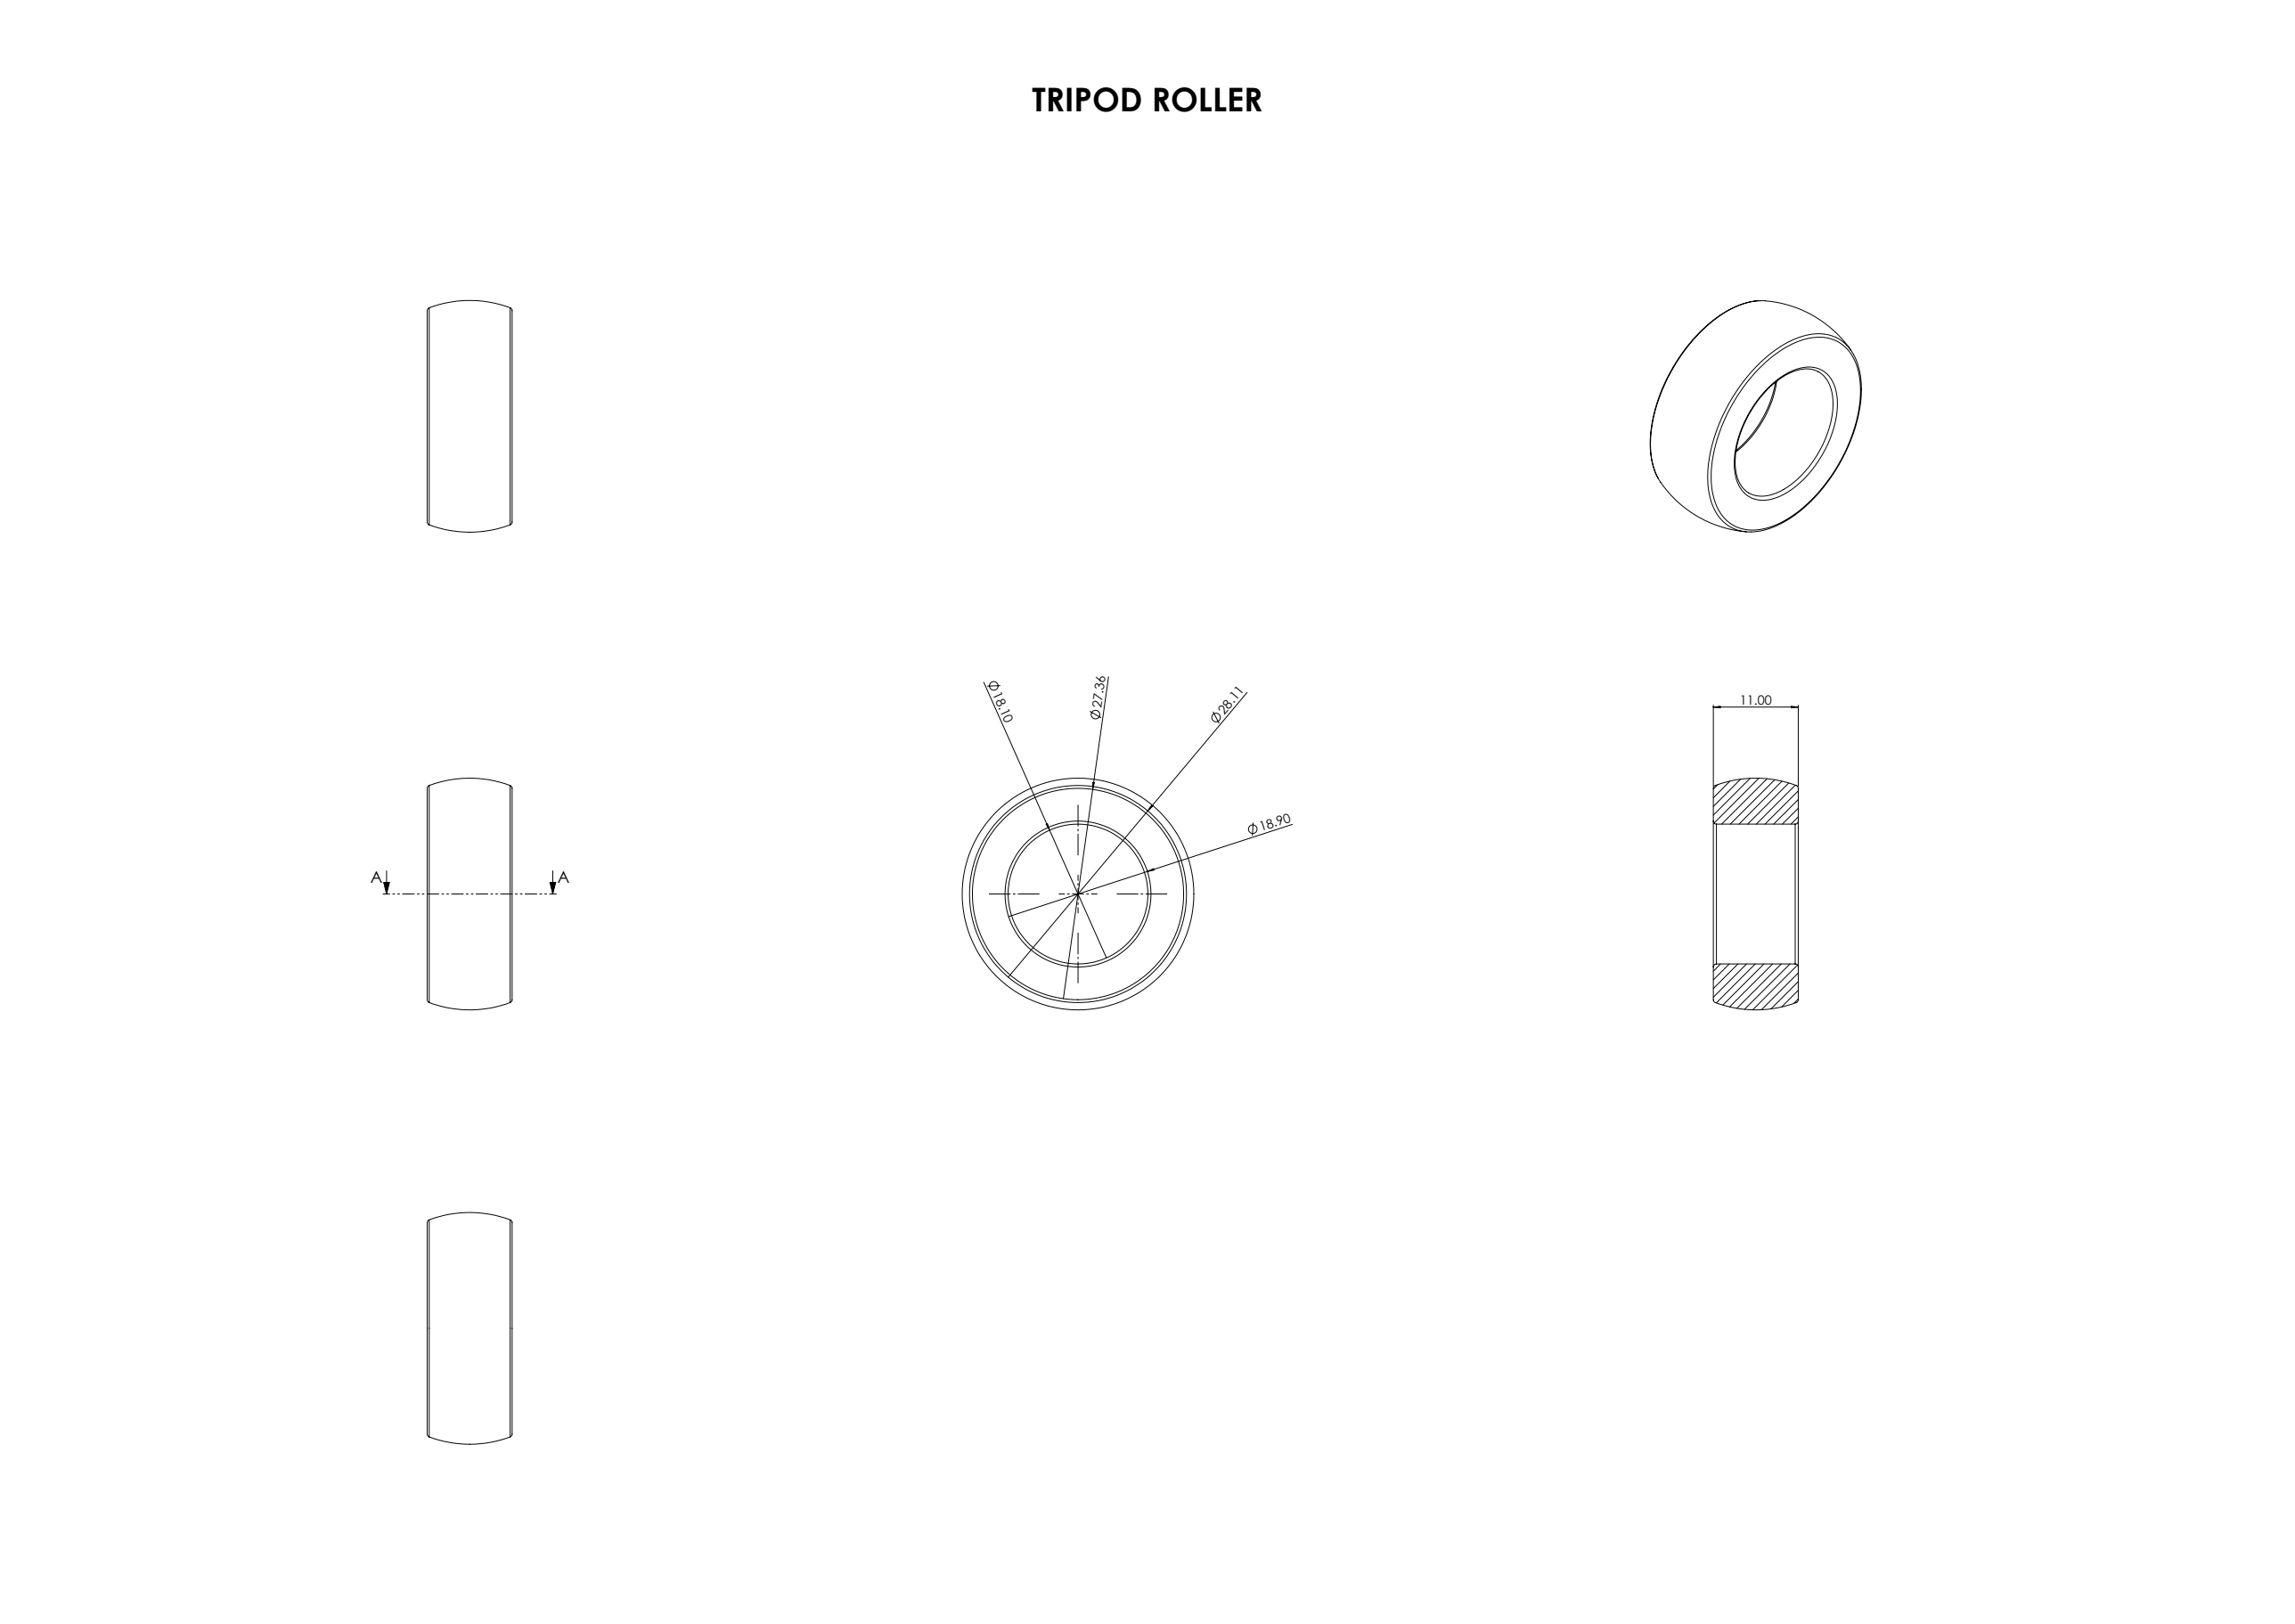
ISO-10303-21;
HEADER;
/* Generated by software containing ST-Developer
 * from STEP Tools, Inc. (www.steptools.com) 
 */

FILE_DESCRIPTION(
/* description */ (''),
/* implementation_level */ '2;1');

FILE_NAME(
/* name */ '15_Tripod_Roller.step',
/* time_stamp */ '2026-10-11T12:57:03-07:00',
/* author */ (''),
/* organization */ (''),
/* preprocessor_version */ 'ST-DEVELOPER v20.2',
/* originating_system */ 'Autodesk Translation Framework v15.15.0.0',
/* authorisation */ '');

FILE_SCHEMA (('AUTOMOTIVE_DESIGN { 1 0 10303 214 3 1 1 }'));
ENDSEC;

DATA;
#10=MECHANICAL_DESIGN_GEOMETRIC_PRESENTATION_REPRESENTATION('',(#270),#90374);
#236=SHAPE_REPRESENTATION_RELATIONSHIP('SRR','None',#90455,#253);
#253=ADVANCED_BREP_SHAPE_REPRESENTATION('',(#287),#90371);
#270=STYLED_ITEM('',(#90673),#287);
#287=MANIFOLD_SOLID_BREP('Body1',#40359);
#573=SPHERICAL_SURFACE('',#45209,15.);
#1031=TOROIDAL_SURFACE('',#45202,13.6802777749576,0.4);
#1032=TOROIDAL_SURFACE('',#45213,9.45,0.4);
#1033=TOROIDAL_SURFACE('',#45220,9.45,0.4);
#1034=TOROIDAL_SURFACE('',#45225,13.6802777749576,0.4);
#1110=FACE_BOUND('',#6986,.T.);
#1111=FACE_BOUND('',#6988,.T.);
#1112=FACE_BOUND('',#6993,.T.);
#1819=PLANE('',#45207);
#1820=PLANE('',#45223);
#4517=FACE_OUTER_BOUND('',#6984,.T.);
#4518=FACE_OUTER_BOUND('',#6985,.T.);
#4519=FACE_OUTER_BOUND('',#6987,.T.);
#4520=FACE_OUTER_BOUND('',#6989,.T.);
#4521=FACE_OUTER_BOUND('',#6990,.T.);
#4522=FACE_OUTER_BOUND('',#6991,.T.);
#4523=FACE_OUTER_BOUND('',#6992,.T.);
#4524=FACE_OUTER_BOUND('',#6994,.T.);
#6984=EDGE_LOOP('',(#37119,#37120,#37121,#37122,#37123));
#6985=EDGE_LOOP('',(#37124));
#6986=EDGE_LOOP('',(#37125));
#6987=EDGE_LOOP('',(#37126,#37127,#37128,#37129,#37130,#37131));
#6988=EDGE_LOOP('',(#37132));
#6989=EDGE_LOOP('',(#37133,#37134,#37135,#37136,#37137));
#6990=EDGE_LOOP('',(#37138,#37139,#37140,#37141,#37142,#37143));
#6991=EDGE_LOOP('',(#37144,#37145,#37146,#37147,#37148));
#6992=EDGE_LOOP('',(#37149));
#6993=EDGE_LOOP('',(#37150));
#6994=EDGE_LOOP('',(#37151,#37152,#37153,#37154));
#9382=CIRCLE('',#45203,14.0550799057784);
#9383=CIRCLE('',#45204,14.0550799057784);
#9384=CIRCLE('',#45205,0.4);
#9385=CIRCLE('',#45206,13.6802777749576);
#9386=CIRCLE('',#45208,9.45);
#9387=CIRCLE('',#45210,15.);
#9388=CIRCLE('',#45211,15.);
#9389=CIRCLE('',#45212,14.0550799057784);
#9390=CIRCLE('',#45214,0.4);
#9391=CIRCLE('',#45215,9.05);
#9392=CIRCLE('',#45216,9.05);
#9393=CIRCLE('',#45218,9.05);
#9394=CIRCLE('',#45219,9.05);
#9395=CIRCLE('',#45221,0.4);
#9396=CIRCLE('',#45222,9.45);
#9397=CIRCLE('',#45224,13.6802777749576);
#9398=CIRCLE('',#45226,0.4);
#12840=LINE('',#90223,#15334);
#15334=VECTOR('',#57118,9.05);
#19037=VERTEX_POINT('',#90195);
#19038=VERTEX_POINT('',#90196);
#19039=VERTEX_POINT('',#90199);
#19040=VERTEX_POINT('',#90203);
#19041=VERTEX_POINT('',#90206);
#19042=VERTEX_POINT('',#90208);
#19043=VERTEX_POINT('',#90210);
#19044=VERTEX_POINT('',#90213);
#19045=VERTEX_POINT('',#90215);
#19046=VERTEX_POINT('',#90219);
#19047=VERTEX_POINT('',#90220);
#19048=VERTEX_POINT('',#90225);
#19049=VERTEX_POINT('',#90229);
#25071=EDGE_CURVE('',#19037,#19038,#9382,.T.);
#25072=EDGE_CURVE('',#19038,#19037,#9383,.T.);
#25073=EDGE_CURVE('',#19037,#19039,#9384,.T.);
#25074=EDGE_CURVE('',#19039,#19039,#9385,.T.);
#25075=EDGE_CURVE('',#19040,#19040,#9386,.T.);
#25076=EDGE_CURVE('',#19041,#19037,#9387,.T.);
#25077=EDGE_CURVE('',#19038,#19042,#9388,.T.);
#25078=EDGE_CURVE('',#19043,#19043,#9389,.T.);
#25079=EDGE_CURVE('',#19040,#19044,#9390,.T.);
#25080=EDGE_CURVE('',#19044,#19045,#9391,.T.);
#25081=EDGE_CURVE('',#19045,#19044,#9392,.T.);
#25082=EDGE_CURVE('',#19046,#19047,#9393,.T.);
#25083=EDGE_CURVE('',#19047,#19046,#9394,.T.);
#25084=EDGE_CURVE('',#19047,#19045,#12840,.T.);
#25085=EDGE_CURVE('',#19046,#19048,#9395,.T.);
#25086=EDGE_CURVE('',#19048,#19048,#9396,.T.);
#25087=EDGE_CURVE('',#19049,#19049,#9397,.T.);
#25088=EDGE_CURVE('',#19049,#19043,#9398,.T.);
#37119=ORIENTED_EDGE('',*,*,#25071,.T.);
#37120=ORIENTED_EDGE('',*,*,#25072,.T.);
#37121=ORIENTED_EDGE('',*,*,#25073,.T.);
#37122=ORIENTED_EDGE('',*,*,#25074,.T.);
#37123=ORIENTED_EDGE('',*,*,#25073,.F.);
#37124=ORIENTED_EDGE('',*,*,#25074,.F.);
#37125=ORIENTED_EDGE('',*,*,#25075,.F.);
#37126=ORIENTED_EDGE('',*,*,#25071,.F.);
#37127=ORIENTED_EDGE('',*,*,#25076,.F.);
#37128=ORIENTED_EDGE('',*,*,#25076,.T.);
#37129=ORIENTED_EDGE('',*,*,#25072,.F.);
#37130=ORIENTED_EDGE('',*,*,#25077,.T.);
#37131=ORIENTED_EDGE('',*,*,#25077,.F.);
#37132=ORIENTED_EDGE('',*,*,#25078,.F.);
#37133=ORIENTED_EDGE('',*,*,#25075,.T.);
#37134=ORIENTED_EDGE('',*,*,#25079,.T.);
#37135=ORIENTED_EDGE('',*,*,#25080,.T.);
#37136=ORIENTED_EDGE('',*,*,#25081,.T.);
#37137=ORIENTED_EDGE('',*,*,#25079,.F.);
#37138=ORIENTED_EDGE('',*,*,#25082,.F.);
#37139=ORIENTED_EDGE('',*,*,#25083,.F.);
#37140=ORIENTED_EDGE('',*,*,#25084,.T.);
#37141=ORIENTED_EDGE('',*,*,#25080,.F.);
#37142=ORIENTED_EDGE('',*,*,#25081,.F.);
#37143=ORIENTED_EDGE('',*,*,#25084,.F.);
#37144=ORIENTED_EDGE('',*,*,#25082,.T.);
#37145=ORIENTED_EDGE('',*,*,#25083,.T.);
#37146=ORIENTED_EDGE('',*,*,#25085,.T.);
#37147=ORIENTED_EDGE('',*,*,#25086,.T.);
#37148=ORIENTED_EDGE('',*,*,#25085,.F.);
#37149=ORIENTED_EDGE('',*,*,#25087,.F.);
#37150=ORIENTED_EDGE('',*,*,#25086,.F.);
#37151=ORIENTED_EDGE('',*,*,#25087,.T.);
#37152=ORIENTED_EDGE('',*,*,#25088,.T.);
#37153=ORIENTED_EDGE('',*,*,#25078,.T.);
#37154=ORIENTED_EDGE('',*,*,#25088,.F.);
#37942=CYLINDRICAL_SURFACE('',#45217,9.05);
#40320=ADVANCED_FACE('',(#4517),#1031,.T.);
#40321=ADVANCED_FACE('',(#4518,#1110),#1819,.T.);
#40322=ADVANCED_FACE('',(#4519,#1111),#573,.T.);
#40323=ADVANCED_FACE('',(#4520),#1032,.T.);
#40324=ADVANCED_FACE('',(#4521),#37942,.F.);
#40325=ADVANCED_FACE('',(#4522),#1033,.T.);
#40326=ADVANCED_FACE('',(#4523,#1112),#1820,.T.);
#40327=ADVANCED_FACE('',(#4524),#1034,.T.);
#40359=CLOSED_SHELL('',(#40320,#40321,#40322,#40323,#40324,#40325,#40326,
#40327));
#45201=AXIS2_PLACEMENT_3D('',#90193,#57080,#57081);
#45202=AXIS2_PLACEMENT_3D('',#90194,#57082,#57083);
#45203=AXIS2_PLACEMENT_3D('',#90197,#57084,#57085);
#45204=AXIS2_PLACEMENT_3D('',#90198,#57086,#57087);
#45205=AXIS2_PLACEMENT_3D('',#90200,#57088,#57089);
#45206=AXIS2_PLACEMENT_3D('',#90201,#57090,#57091);
#45207=AXIS2_PLACEMENT_3D('',#90202,#57092,#57093);
#45208=AXIS2_PLACEMENT_3D('',#90204,#57094,#57095);
#45209=AXIS2_PLACEMENT_3D('',#90205,#57096,#57097);
#45210=AXIS2_PLACEMENT_3D('',#90207,#57098,#57099);
#45211=AXIS2_PLACEMENT_3D('',#90209,#57100,#57101);
#45212=AXIS2_PLACEMENT_3D('',#90211,#57102,#57103);
#45213=AXIS2_PLACEMENT_3D('',#90212,#57104,#57105);
#45214=AXIS2_PLACEMENT_3D('',#90214,#57106,#57107);
#45215=AXIS2_PLACEMENT_3D('',#90216,#57108,#57109);
#45216=AXIS2_PLACEMENT_3D('',#90217,#57110,#57111);
#45217=AXIS2_PLACEMENT_3D('',#90218,#57112,#57113);
#45218=AXIS2_PLACEMENT_3D('',#90221,#57114,#57115);
#45219=AXIS2_PLACEMENT_3D('',#90222,#57116,#57117);
#45220=AXIS2_PLACEMENT_3D('',#90224,#57119,#57120);
#45221=AXIS2_PLACEMENT_3D('',#90226,#57121,#57122);
#45222=AXIS2_PLACEMENT_3D('',#90227,#57123,#57124);
#45223=AXIS2_PLACEMENT_3D('',#90228,#57125,#57126);
#45224=AXIS2_PLACEMENT_3D('',#90230,#57127,#57128);
#45225=AXIS2_PLACEMENT_3D('',#90231,#57129,#57130);
#45226=AXIS2_PLACEMENT_3D('',#90232,#57131,#57132);
#57080=DIRECTION('axis',(0.,0.,1.));
#57081=DIRECTION('refdir',(1.,0.,0.));
#57082=DIRECTION('center_axis',(1.,0.,0.));
#57083=DIRECTION('ref_axis',(0.,0.,-1.));
#57084=DIRECTION('center_axis',(-1.,0.,0.));
#57085=DIRECTION('ref_axis',(0.,-1.,1.83697019872103E-16));
#57086=DIRECTION('center_axis',(-1.,0.,0.));
#57087=DIRECTION('ref_axis',(0.,-1.,1.83697019872103E-16));
#57088=DIRECTION('center_axis',(0.,-1.,-1.22464679914735E-16));
#57089=DIRECTION('ref_axis',(0.,-1.22464679914735E-16,1.));
#57090=DIRECTION('center_axis',(1.,0.,0.));
#57091=DIRECTION('ref_axis',(0.,-1.,1.83697019872103E-16));
#57092=DIRECTION('center_axis',(-1.,0.,0.));
#57093=DIRECTION('ref_axis',(0.,0.,1.));
#57094=DIRECTION('center_axis',(-1.,0.,0.));
#57095=DIRECTION('ref_axis',(0.,-1.,1.83697019872103E-16));
#57096=DIRECTION('center_axis',(6.12323399573677E-17,0.,1.));
#57097=DIRECTION('ref_axis',(1.,0.,0.));
#57098=DIRECTION('center_axis',(1.22464679914735E-16,-1.,0.));
#57099=DIRECTION('ref_axis',(-1.,-1.22464679914735E-16,0.));
#57100=DIRECTION('center_axis',(1.22464679914735E-16,-1.,0.));
#57101=DIRECTION('ref_axis',(-1.,-1.22464679914735E-16,0.));
#57102=DIRECTION('center_axis',(1.,0.,0.));
#57103=DIRECTION('ref_axis',(0.,-1.,1.83697019872103E-16));
#57104=DIRECTION('center_axis',(1.,0.,0.));
#57105=DIRECTION('ref_axis',(0.,0.,-1.));
#57106=DIRECTION('center_axis',(0.,-1.,-1.22464679914735E-16));
#57107=DIRECTION('ref_axis',(0.,-1.22464679914735E-16,1.));
#57108=DIRECTION('center_axis',(1.,0.,0.));
#57109=DIRECTION('ref_axis',(0.,-1.,1.83697019872103E-16));
#57110=DIRECTION('center_axis',(1.,0.,0.));
#57111=DIRECTION('ref_axis',(0.,-1.,1.83697019872103E-16));
#57112=DIRECTION('center_axis',(1.,0.,0.));
#57113=DIRECTION('ref_axis',(0.,1.,0.));
#57114=DIRECTION('center_axis',(-1.,0.,0.));
#57115=DIRECTION('ref_axis',(0.,-1.,1.83697019872103E-16));
#57116=DIRECTION('center_axis',(-1.,0.,0.));
#57117=DIRECTION('ref_axis',(0.,-1.,1.83697019872103E-16));
#57118=DIRECTION('',(-1.,0.,0.));
#57119=DIRECTION('center_axis',(1.,0.,0.));
#57120=DIRECTION('ref_axis',(0.,0.,-1.));
#57121=DIRECTION('center_axis',(0.,-1.,-1.22464679914735E-16));
#57122=DIRECTION('ref_axis',(0.,-1.22464679914735E-16,1.));
#57123=DIRECTION('center_axis',(1.,0.,0.));
#57124=DIRECTION('ref_axis',(0.,-1.,1.83697019872103E-16));
#57125=DIRECTION('center_axis',(1.,0.,0.));
#57126=DIRECTION('ref_axis',(0.,0.,-1.));
#57127=DIRECTION('center_axis',(-1.,0.,0.));
#57128=DIRECTION('ref_axis',(0.,-1.,1.83697019872103E-16));
#57129=DIRECTION('center_axis',(1.,0.,0.));
#57130=DIRECTION('ref_axis',(0.,0.,-1.));
#57131=DIRECTION('center_axis',(0.,-1.,-1.22464679914735E-16));
#57132=DIRECTION('ref_axis',(0.,-1.22464679914735E-16,1.));
#90193=CARTESIAN_POINT('',(0.,0.,0.));
#90194=CARTESIAN_POINT('Origin',(-5.1,-2.22044604925031E-15,0.));
#90195=CARTESIAN_POINT('',(-5.23972602739726,-3.94169691108749E-15,14.0550799057784));
#90196=CARTESIAN_POINT('',(-5.23972602739726,-2.86212742003643E-15,-14.0550799057784));
#90197=CARTESIAN_POINT('Origin',(-5.23972602739726,-2.22044604925031E-15,
0.));
#90198=CARTESIAN_POINT('Origin',(-5.23972602739726,-2.22044604925031E-15,
0.));
#90199=CARTESIAN_POINT('',(-5.5,-3.89579688810517E-15,13.6802777749576));
#90200=CARTESIAN_POINT('Origin',(-5.1,-3.89579688810517E-15,13.6802777749576));
#90201=CARTESIAN_POINT('Origin',(-5.5,-2.22044604925031E-15,0.));
#90202=CARTESIAN_POINT('Origin',(-5.5,13.9552857369529,0.));
#90203=CARTESIAN_POINT('',(-5.5,-1.15729122519425E-15,9.45));
#90204=CARTESIAN_POINT('Origin',(-5.5,0.,0.));
#90205=CARTESIAN_POINT('Origin',(0.,-2.22044604925031E-15,0.));
#90206=CARTESIAN_POINT('',(-9.18485099360515E-16,-2.22044604925031E-15,
15.));
#90207=CARTESIAN_POINT('Origin',(0.,-2.22044604925031E-15,0.));
#90208=CARTESIAN_POINT('',(-9.18485099360515E-16,-2.22044604925031E-15,
-15.));
#90209=CARTESIAN_POINT('Origin',(0.,-2.22044604925031E-15,0.));
#90210=CARTESIAN_POINT('',(5.23972602739726,-3.94169691108749E-15,14.0550799057784));
#90211=CARTESIAN_POINT('Origin',(5.23972602739726,-2.22044604925031E-15,
0.));
#90212=CARTESIAN_POINT('Origin',(-5.1,0.,0.));
#90213=CARTESIAN_POINT('',(-5.1,-1.10830535322835E-15,9.05));
#90214=CARTESIAN_POINT('Origin',(-5.1,-1.15729122519425E-15,9.45));
#90215=CARTESIAN_POINT('',(-5.1,-9.05,-1.10830535322835E-15));
#90216=CARTESIAN_POINT('Origin',(-5.1,0.,0.));
#90217=CARTESIAN_POINT('Origin',(-5.1,0.,0.));
#90218=CARTESIAN_POINT('Origin',(0.,0.,0.));
#90219=CARTESIAN_POINT('',(5.1,-1.10830535322835E-15,9.05));
#90220=CARTESIAN_POINT('',(5.1,-9.05,-1.10830535322835E-15));
#90221=CARTESIAN_POINT('Origin',(5.1,0.,0.));
#90222=CARTESIAN_POINT('Origin',(5.1,0.,0.));
#90223=CARTESIAN_POINT('',(0.,-9.05,-1.10830535322835E-15));
#90224=CARTESIAN_POINT('Origin',(5.1,0.,0.));
#90225=CARTESIAN_POINT('',(5.5,-1.15729122519425E-15,9.45));
#90226=CARTESIAN_POINT('Origin',(5.1,-1.15729122519425E-15,9.45));
#90227=CARTESIAN_POINT('Origin',(5.5,0.,0.));
#90228=CARTESIAN_POINT('Origin',(5.5,9.05,0.));
#90229=CARTESIAN_POINT('',(5.5,-3.89579688810517E-15,13.6802777749576));
#90230=CARTESIAN_POINT('Origin',(5.5,-2.22044604925031E-15,0.));
#90231=CARTESIAN_POINT('Origin',(5.1,-2.22044604925031E-15,0.));
#90232=CARTESIAN_POINT('Origin',(5.1,-3.89579688810517E-15,13.6802777749576));
#90352=UNCERTAINTY_MEASURE_WITH_UNIT(LENGTH_MEASURE(0.01),#90375,
'DISTANCE_ACCURACY_VALUE',
'Maximum model space distance between geometric entities at asserted c
onnectivities');
#90355=UNCERTAINTY_MEASURE_WITH_UNIT(LENGTH_MEASURE(0.01),#90375,
'DISTANCE_ACCURACY_VALUE',
'Maximum model space distance between geometric entities at asserted c
onnectivities');
#90371=(
GEOMETRIC_REPRESENTATION_CONTEXT(3)
GLOBAL_UNCERTAINTY_ASSIGNED_CONTEXT((#90352))
GLOBAL_UNIT_ASSIGNED_CONTEXT((#90375,#90377,#90378))
REPRESENTATION_CONTEXT('','3D')
);
#90374=(
GEOMETRIC_REPRESENTATION_CONTEXT(3)
GLOBAL_UNCERTAINTY_ASSIGNED_CONTEXT((#90355))
GLOBAL_UNIT_ASSIGNED_CONTEXT((#90375,#90377,#90378))
REPRESENTATION_CONTEXT('','3D')
);
#90375=(
LENGTH_UNIT()
NAMED_UNIT(*)
SI_UNIT(.MILLI.,.METRE.)
);
#90377=(
NAMED_UNIT(*)
PLANE_ANGLE_UNIT()
SI_UNIT($,.RADIAN.)
);
#90378=(
NAMED_UNIT(*)
SI_UNIT($,.STERADIAN.)
SOLID_ANGLE_UNIT()
);
#90394=SHAPE_DEFINITION_REPRESENTATION(#90412,#90455);
#90412=PRODUCT_DEFINITION_SHAPE('',$,#90474);
#90455=SHAPE_REPRESENTATION('',(#45201),#90371);
#90458=PRODUCT_DEFINITION_CONTEXT('part definition',#90514,'design');
#90474=PRODUCT_DEFINITION('2026-10-11-12-53-15-782','15_Tripod_Roller',
#90492,#90458);
#90492=PRODUCT_DEFINITION_FORMATION('',$,#90531);
#90514=APPLICATION_CONTEXT(
'Core Data for Automotive Mechanical Design Process');
#90515=PRODUCT_CONTEXT('part definition',#90514,'mechanical');
#90531=PRODUCT('2026-10-11-12-53-15-782','15_Tripod_Roller',$,(#90515));
#90667=COLOUR_RGB('Light Blue',0.38,0.62,0.78);
#90668=FILL_AREA_STYLE_COLOUR('',#90667);
#90669=FILL_AREA_STYLE('',(#90668));
#90670=SURFACE_STYLE_FILL_AREA(#90669);
#90671=SURFACE_SIDE_STYLE('',(#90670));
#90672=SURFACE_STYLE_USAGE(.BOTH.,#90671);
#90673=PRESENTATION_STYLE_ASSIGNMENT((#90672));
ENDSEC;
END-ISO-10303-21;
